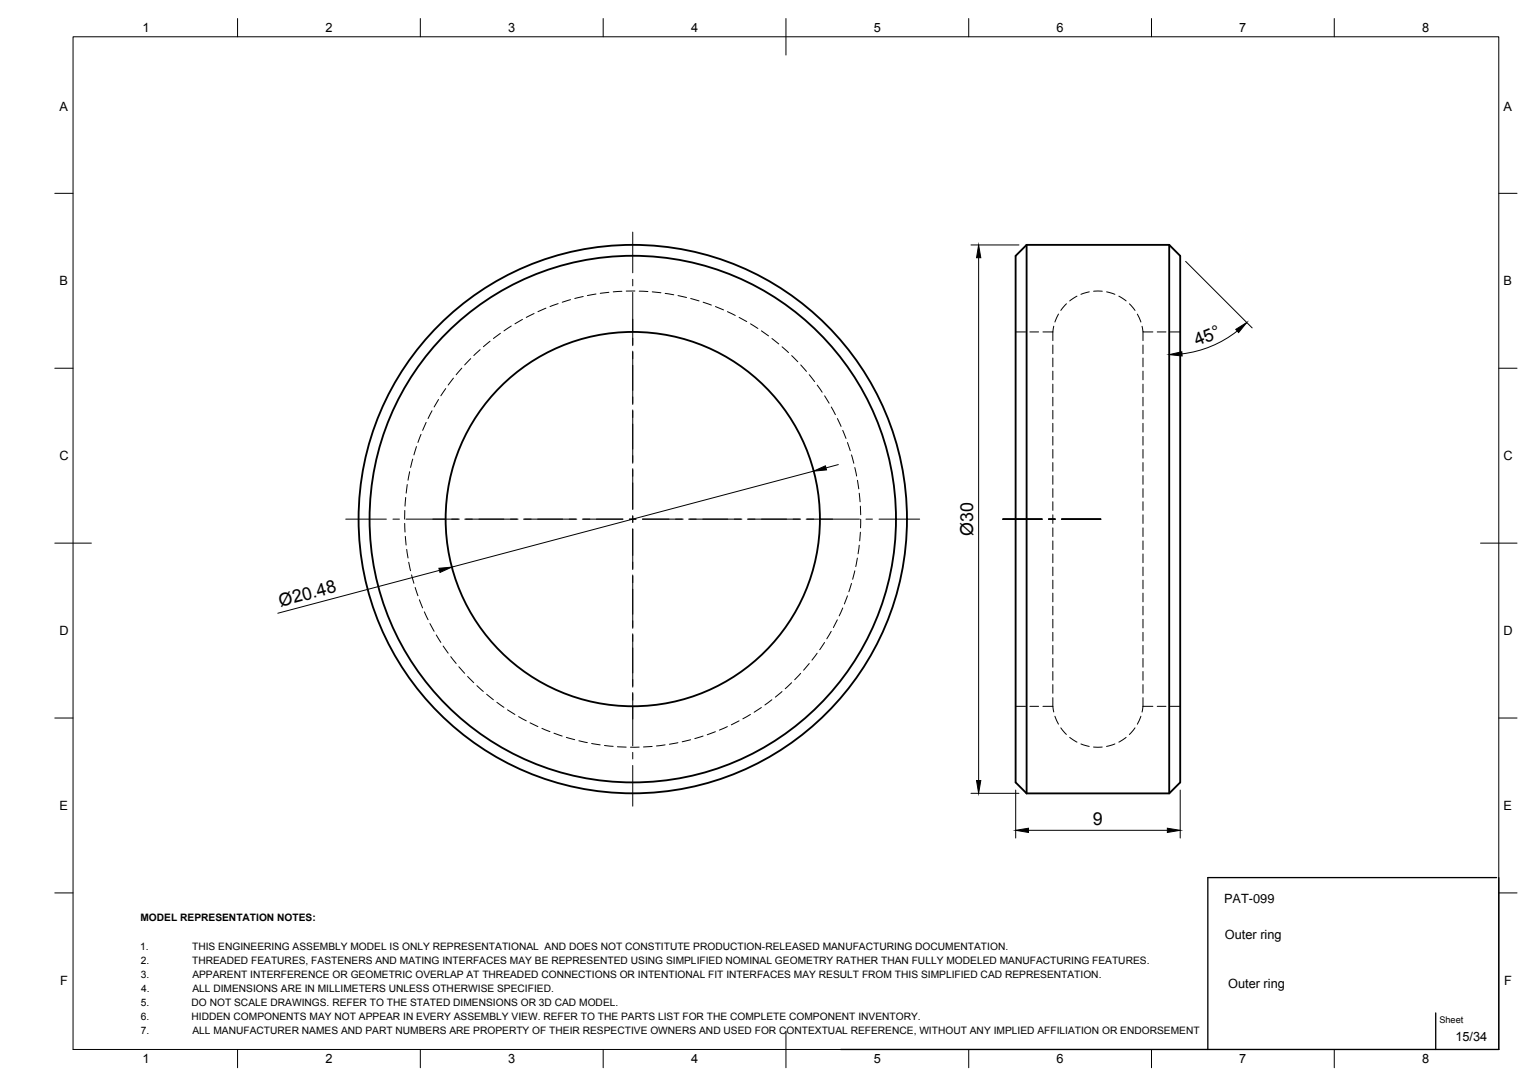
ISO-10303-21;
HEADER;
/* Generated by software containing ST-Developer
 * from STEP Tools, Inc. (www.steptools.com) 
 */

FILE_DESCRIPTION(
/* description */ ('PAT-099'),
/* implementation_level */ '2;1');

FILE_NAME(
/* name */ 'Outer ring.step',
/* time_stamp */ '2026-10-29T17:25:42-07:00',
/* author */ (''),
/* organization */ (''),
/* preprocessor_version */ 'ST-DEVELOPER v20.2',
/* originating_system */ 'Autodesk Translation Framework v15.17.0.0',
/* authorisation */ '');

FILE_SCHEMA (('AUTOMOTIVE_DESIGN { 1 0 10303 214 3 1 1 }'));
ENDSEC;

DATA;
#10=MECHANICAL_DESIGN_GEOMETRIC_PRESENTATION_REPRESENTATION('',(#358),#11035);
#28=TOROIDAL_SURFACE('',#5524,1.,0.247676);
#38=CONICAL_SURFACE('',#5535,1.47,0.785398163397449);
#39=CONICAL_SURFACE('',#5539,1.47,0.785398163397449);
#308=SHAPE_REPRESENTATION_RELATIONSHIP('SRR','None',#11181,#333);
#333=ADVANCED_BREP_SHAPE_REPRESENTATION('',(#389),#11031);
#358=STYLED_ITEM('',(#11386),#389);
#389=MANIFOLD_SOLID_BREP('Body1',#4728);
#516=FACE_BOUND('',#1296,.T.);
#517=FACE_BOUND('',#1301,.T.);
#644=PLANE('',#5532);
#645=PLANE('',#5541);
#897=FACE_OUTER_BOUND('',#1293,.T.);
#898=FACE_OUTER_BOUND('',#1294,.T.);
#899=FACE_OUTER_BOUND('',#1295,.T.);
#900=FACE_OUTER_BOUND('',#1297,.T.);
#901=FACE_OUTER_BOUND('',#1298,.T.);
#902=FACE_OUTER_BOUND('',#1299,.T.);
#903=FACE_OUTER_BOUND('',#1300,.T.);
#904=FACE_OUTER_BOUND('',#1302,.T.);
#1293=EDGE_LOOP('',(#4129,#4130,#4131,#4132,#4133,#4134));
#1294=EDGE_LOOP('',(#4135,#4136,#4137,#4138,#4139));
#1295=EDGE_LOOP('',(#4140));
#1296=EDGE_LOOP('',(#4141));
#1297=EDGE_LOOP('',(#4142,#4143,#4144,#4145));
#1298=EDGE_LOOP('',(#4146,#4147,#4148,#4149));
#1299=EDGE_LOOP('',(#4150,#4151,#4152,#4153));
#1300=EDGE_LOOP('',(#4154));
#1301=EDGE_LOOP('',(#4155));
#1302=EDGE_LOOP('',(#4156,#4157,#4158,#4159,#4160));
#1584=LINE('',#10402,#1836);
#1585=LINE('',#10411,#1837);
#1586=LINE('',#10415,#1838);
#1587=LINE('',#10419,#1839);
#1588=LINE('',#10422,#1840);
#1836=VECTOR('',#6941,1.023815);
#1837=VECTOR('',#6952,1.47);
#1838=VECTOR('',#6957,1.5);
#1839=VECTOR('',#6962,1.47);
#1840=VECTOR('',#6967,1.023815);
#2077=CIRCLE('',#5525,1.023815);
#2078=CIRCLE('',#5526,1.023815);
#2079=CIRCLE('',#5527,0.247676);
#2080=CIRCLE('',#5528,1.023815);
#2081=CIRCLE('',#5529,1.023815);
#2082=CIRCLE('',#5531,1.023815);
#2083=CIRCLE('',#5533,1.44);
#2084=CIRCLE('',#5534,1.023815);
#2085=CIRCLE('',#5536,1.5);
#2086=CIRCLE('',#5538,1.5);
#2087=CIRCLE('',#5540,1.44);
#2472=VERTEX_POINT('',#10390);
#2473=VERTEX_POINT('',#10391);
#2474=VERTEX_POINT('',#10394);
#2475=VERTEX_POINT('',#10396);
#2476=VERTEX_POINT('',#10400);
#2477=VERTEX_POINT('',#10404);
#2478=VERTEX_POINT('',#10406);
#2479=VERTEX_POINT('',#10409);
#2480=VERTEX_POINT('',#10413);
#2481=VERTEX_POINT('',#10417);
#3041=EDGE_CURVE('',#2472,#2473,#2077,.T.);
#3042=EDGE_CURVE('',#2473,#2472,#2078,.T.);
#3043=EDGE_CURVE('',#2473,#2474,#2079,.T.);
#3044=EDGE_CURVE('',#2475,#2474,#2080,.T.);
#3045=EDGE_CURVE('',#2474,#2475,#2081,.T.);
#3046=EDGE_CURVE('',#2476,#2476,#2082,.T.);
#3047=EDGE_CURVE('',#2476,#2475,#1584,.T.);
#3048=EDGE_CURVE('',#2477,#2477,#2083,.T.);
#3049=EDGE_CURVE('',#2478,#2478,#2084,.T.);
#3050=EDGE_CURVE('',#2479,#2479,#2085,.T.);
#3051=EDGE_CURVE('',#2479,#2477,#1585,.T.);
#3052=EDGE_CURVE('',#2480,#2480,#2086,.T.);
#3053=EDGE_CURVE('',#2480,#2479,#1586,.T.);
#3054=EDGE_CURVE('',#2481,#2481,#2087,.T.);
#3055=EDGE_CURVE('',#2481,#2480,#1587,.T.);
#3056=EDGE_CURVE('',#2472,#2478,#1588,.T.);
#4129=ORIENTED_EDGE('',*,*,#3041,.F.);
#4130=ORIENTED_EDGE('',*,*,#3042,.F.);
#4131=ORIENTED_EDGE('',*,*,#3043,.T.);
#4132=ORIENTED_EDGE('',*,*,#3044,.F.);
#4133=ORIENTED_EDGE('',*,*,#3045,.F.);
#4134=ORIENTED_EDGE('',*,*,#3043,.F.);
#4135=ORIENTED_EDGE('',*,*,#3046,.T.);
#4136=ORIENTED_EDGE('',*,*,#3047,.T.);
#4137=ORIENTED_EDGE('',*,*,#3044,.T.);
#4138=ORIENTED_EDGE('',*,*,#3045,.T.);
#4139=ORIENTED_EDGE('',*,*,#3047,.F.);
#4140=ORIENTED_EDGE('',*,*,#3048,.F.);
#4141=ORIENTED_EDGE('',*,*,#3049,.T.);
#4142=ORIENTED_EDGE('',*,*,#3050,.F.);
#4143=ORIENTED_EDGE('',*,*,#3051,.T.);
#4144=ORIENTED_EDGE('',*,*,#3048,.T.);
#4145=ORIENTED_EDGE('',*,*,#3051,.F.);
#4146=ORIENTED_EDGE('',*,*,#3052,.F.);
#4147=ORIENTED_EDGE('',*,*,#3053,.T.);
#4148=ORIENTED_EDGE('',*,*,#3050,.T.);
#4149=ORIENTED_EDGE('',*,*,#3053,.F.);
#4150=ORIENTED_EDGE('',*,*,#3054,.F.);
#4151=ORIENTED_EDGE('',*,*,#3055,.T.);
#4152=ORIENTED_EDGE('',*,*,#3052,.T.);
#4153=ORIENTED_EDGE('',*,*,#3055,.F.);
#4154=ORIENTED_EDGE('',*,*,#3054,.T.);
#4155=ORIENTED_EDGE('',*,*,#3046,.F.);
#4156=ORIENTED_EDGE('',*,*,#3041,.T.);
#4157=ORIENTED_EDGE('',*,*,#3042,.T.);
#4158=ORIENTED_EDGE('',*,*,#3056,.T.);
#4159=ORIENTED_EDGE('',*,*,#3049,.F.);
#4160=ORIENTED_EDGE('',*,*,#3056,.F.);
#4415=CYLINDRICAL_SURFACE('',#5530,1.023815);
#4416=CYLINDRICAL_SURFACE('',#5537,1.5);
#4417=CYLINDRICAL_SURFACE('',#5542,1.023815);
#4662=ADVANCED_FACE('',(#897),#28,.F.);
#4663=ADVANCED_FACE('',(#898),#4415,.F.);
#4664=ADVANCED_FACE('',(#899,#516),#644,.T.);
#4665=ADVANCED_FACE('',(#900),#38,.T.);
#4666=ADVANCED_FACE('',(#901),#4416,.T.);
#4667=ADVANCED_FACE('',(#902),#39,.T.);
#4668=ADVANCED_FACE('',(#903,#517),#645,.T.);
#4669=ADVANCED_FACE('',(#904),#4417,.F.);
#4728=CLOSED_SHELL('',(#4662,#4663,#4664,#4665,#4666,#4667,#4668,#4669));
#5523=AXIS2_PLACEMENT_3D('',#10388,#6923,#6924);
#5524=AXIS2_PLACEMENT_3D('',#10389,#6925,#6926);
#5525=AXIS2_PLACEMENT_3D('',#10392,#6927,#6928);
#5526=AXIS2_PLACEMENT_3D('',#10393,#6929,#6930);
#5527=AXIS2_PLACEMENT_3D('',#10395,#6931,#6932);
#5528=AXIS2_PLACEMENT_3D('',#10397,#6933,#6934);
#5529=AXIS2_PLACEMENT_3D('',#10398,#6935,#6936);
#5530=AXIS2_PLACEMENT_3D('',#10399,#6937,#6938);
#5531=AXIS2_PLACEMENT_3D('',#10401,#6939,#6940);
#5532=AXIS2_PLACEMENT_3D('',#10403,#6942,#6943);
#5533=AXIS2_PLACEMENT_3D('',#10405,#6944,#6945);
#5534=AXIS2_PLACEMENT_3D('',#10407,#6946,#6947);
#5535=AXIS2_PLACEMENT_3D('',#10408,#6948,#6949);
#5536=AXIS2_PLACEMENT_3D('',#10410,#6950,#6951);
#5537=AXIS2_PLACEMENT_3D('',#10412,#6953,#6954);
#5538=AXIS2_PLACEMENT_3D('',#10414,#6955,#6956);
#5539=AXIS2_PLACEMENT_3D('',#10416,#6958,#6959);
#5540=AXIS2_PLACEMENT_3D('',#10418,#6960,#6961);
#5541=AXIS2_PLACEMENT_3D('',#10420,#6963,#6964);
#5542=AXIS2_PLACEMENT_3D('',#10421,#6965,#6966);
#6923=DIRECTION('axis',(0.,0.,1.));
#6924=DIRECTION('refdir',(1.,0.,0.));
#6925=DIRECTION('center_axis',(0.,-1.,0.));
#6926=DIRECTION('ref_axis',(0.,0.,-1.));
#6927=DIRECTION('center_axis',(0.,-1.,0.));
#6928=DIRECTION('ref_axis',(1.,0.,0.));
#6929=DIRECTION('center_axis',(0.,-1.,0.));
#6930=DIRECTION('ref_axis',(1.,0.,0.));
#6931=DIRECTION('center_axis',(1.,0.,1.22464679914735E-16));
#6932=DIRECTION('ref_axis',(-1.22464679914735E-16,0.,1.));
#6933=DIRECTION('center_axis',(0.,1.,0.));
#6934=DIRECTION('ref_axis',(1.,0.,0.));
#6935=DIRECTION('center_axis',(0.,1.,0.));
#6936=DIRECTION('ref_axis',(1.,0.,0.));
#6937=DIRECTION('center_axis',(0.,-1.,0.));
#6938=DIRECTION('ref_axis',(1.,0.,0.));
#6939=DIRECTION('center_axis',(0.,-1.,0.));
#6940=DIRECTION('ref_axis',(1.,0.,0.));
#6941=DIRECTION('',(0.,1.,0.));
#6942=DIRECTION('center_axis',(0.,1.,0.));
#6943=DIRECTION('ref_axis',(0.,0.,1.));
#6944=DIRECTION('center_axis',(0.,-1.,0.));
#6945=DIRECTION('ref_axis',(1.,0.,0.));
#6946=DIRECTION('center_axis',(0.,-1.,0.));
#6947=DIRECTION('ref_axis',(1.,0.,0.));
#6948=DIRECTION('center_axis',(0.,-1.,0.));
#6949=DIRECTION('ref_axis',(1.,0.,0.));
#6950=DIRECTION('center_axis',(0.,-1.,0.));
#6951=DIRECTION('ref_axis',(1.,0.,0.));
#6952=DIRECTION('',(0.707106781186548,0.707106781186547,8.65956056235494E-17));
#6953=DIRECTION('center_axis',(0.,-1.,0.));
#6954=DIRECTION('ref_axis',(1.,0.,0.));
#6955=DIRECTION('center_axis',(0.,-1.,0.));
#6956=DIRECTION('ref_axis',(1.,0.,0.));
#6957=DIRECTION('',(0.,1.,0.));
#6958=DIRECTION('center_axis',(0.,1.,0.));
#6959=DIRECTION('ref_axis',(1.,0.,0.));
#6960=DIRECTION('center_axis',(0.,-1.,0.));
#6961=DIRECTION('ref_axis',(1.,0.,0.));
#6962=DIRECTION('',(-0.707106781186548,0.707106781186547,-8.65956056235494E-17));
#6963=DIRECTION('center_axis',(0.,-1.,0.));
#6964=DIRECTION('ref_axis',(0.,0.,-1.));
#6965=DIRECTION('center_axis',(0.,-1.,0.));
#6966=DIRECTION('ref_axis',(1.,0.,0.));
#6967=DIRECTION('',(0.,1.,0.));
#10388=CARTESIAN_POINT('',(0.,0.,0.));
#10389=CARTESIAN_POINT('Origin',(0.,0.,0.));
#10390=CARTESIAN_POINT('',(-1.023815,0.246528389340863,-1.25381176266905E-16));
#10391=CARTESIAN_POINT('',(-1.25381176266905E-16,0.246528389340863,1.023815));
#10392=CARTESIAN_POINT('Origin',(0.,0.246528389340863,0.));
#10393=CARTESIAN_POINT('Origin',(0.,0.246528389340863,0.));
#10394=CARTESIAN_POINT('',(-1.25381176266905E-16,-0.246528389340863,1.023815));
#10395=CARTESIAN_POINT('Origin',(-1.22464679914735E-16,0.,1.));
#10396=CARTESIAN_POINT('',(-1.023815,-0.246528389340863,1.25381176266905E-16));
#10397=CARTESIAN_POINT('Origin',(0.,-0.246528389340863,0.));
#10398=CARTESIAN_POINT('Origin',(0.,-0.246528389340863,0.));
#10399=CARTESIAN_POINT('Origin',(0.,0.,0.));
#10400=CARTESIAN_POINT('',(-1.023815,-0.45,-1.25381176266905E-16));
#10401=CARTESIAN_POINT('Origin',(0.,-0.45,0.));
#10402=CARTESIAN_POINT('',(-1.023815,0.,-1.25381176266905E-16));
#10403=CARTESIAN_POINT('Origin',(1.44,0.45,0.));
#10404=CARTESIAN_POINT('',(-1.44,0.45,-1.76349139077219E-16));
#10405=CARTESIAN_POINT('Origin',(0.,0.45,0.));
#10406=CARTESIAN_POINT('',(-1.023815,0.45,-1.25381176266905E-16));
#10407=CARTESIAN_POINT('Origin',(0.,0.45,0.));
#10408=CARTESIAN_POINT('Origin',(0.,0.42,0.));
#10409=CARTESIAN_POINT('',(-1.5,0.39,-1.83697019872103E-16));
#10410=CARTESIAN_POINT('Origin',(0.,0.39,0.));
#10411=CARTESIAN_POINT('',(-1.47,0.42,-1.80023079474661E-16));
#10412=CARTESIAN_POINT('Origin',(0.,0.,0.));
#10413=CARTESIAN_POINT('',(-1.5,-0.39,-1.83697019872103E-16));
#10414=CARTESIAN_POINT('Origin',(0.,-0.39,0.));
#10415=CARTESIAN_POINT('',(-1.5,0.,-1.83697019872103E-16));
#10416=CARTESIAN_POINT('Origin',(0.,-0.42,0.));
#10417=CARTESIAN_POINT('',(-1.44,-0.45,-1.76349139077219E-16));
#10418=CARTESIAN_POINT('Origin',(0.,-0.45,0.));
#10419=CARTESIAN_POINT('',(-1.47,-0.42,-1.80023079474661E-16));
#10420=CARTESIAN_POINT('Origin',(1.023815,-0.45,0.));
#10421=CARTESIAN_POINT('Origin',(0.,0.,0.));
#10422=CARTESIAN_POINT('',(-1.023815,0.,-1.25381176266905E-16));
#10998=UNCERTAINTY_MEASURE_WITH_UNIT(LENGTH_MEASURE(0.001),#11036,
'DISTANCE_ACCURACY_VALUE',
'Maximum model space distance between geometric entities at asserted c
onnectivities');
#11002=UNCERTAINTY_MEASURE_WITH_UNIT(LENGTH_MEASURE(0.001),#11036,
'DISTANCE_ACCURACY_VALUE',
'Maximum model space distance between geometric entities at asserted c
onnectivities');
#11031=(
GEOMETRIC_REPRESENTATION_CONTEXT(3)
GLOBAL_UNCERTAINTY_ASSIGNED_CONTEXT((#10998))
GLOBAL_UNIT_ASSIGNED_CONTEXT((#11036,#11038,#11039))
REPRESENTATION_CONTEXT('','3D')
);
#11035=(
GEOMETRIC_REPRESENTATION_CONTEXT(3)
GLOBAL_UNCERTAINTY_ASSIGNED_CONTEXT((#11002))
GLOBAL_UNIT_ASSIGNED_CONTEXT((#11036,#11038,#11039))
REPRESENTATION_CONTEXT('','3D')
);
#11036=(
LENGTH_UNIT()
NAMED_UNIT(*)
SI_UNIT(.CENTI.,.METRE.)
);
#11038=(
NAMED_UNIT(*)
PLANE_ANGLE_UNIT()
SI_UNIT($,.RADIAN.)
);
#11039=(
NAMED_UNIT(*)
SI_UNIT($,.STERADIAN.)
SOLID_ANGLE_UNIT()
);
#11068=SHAPE_DEFINITION_REPRESENTATION(#11112,#11181);
#11112=PRODUCT_DEFINITION_SHAPE('',$,#11214);
#11181=SHAPE_REPRESENTATION('',(#5523),#11031);
#11185=PRODUCT_DEFINITION_CONTEXT('part definition',#11283,'design');
#11214=PRODUCT_DEFINITION('Outer ring','Outer ring',#11246,#11185);
#11246=PRODUCT_DEFINITION_FORMATION('',$,#11313);
#11283=APPLICATION_CONTEXT(
'Core Data for Automotive Mechanical Design Process');
#11284=PRODUCT_CONTEXT('part definition',#11283,'mechanical');
#11313=PRODUCT('Outer ring','Outer ring','Outer ring',(#11284));
#11380=COLOUR_RGB('Grey',0.48,0.52,0.57);
#11381=FILL_AREA_STYLE_COLOUR('',#11380);
#11382=FILL_AREA_STYLE('',(#11381));
#11383=SURFACE_STYLE_FILL_AREA(#11382);
#11384=SURFACE_SIDE_STYLE('',(#11383));
#11385=SURFACE_STYLE_USAGE(.BOTH.,#11384);
#11386=PRESENTATION_STYLE_ASSIGNMENT((#11385));
ENDSEC;
END-ISO-10303-21;
